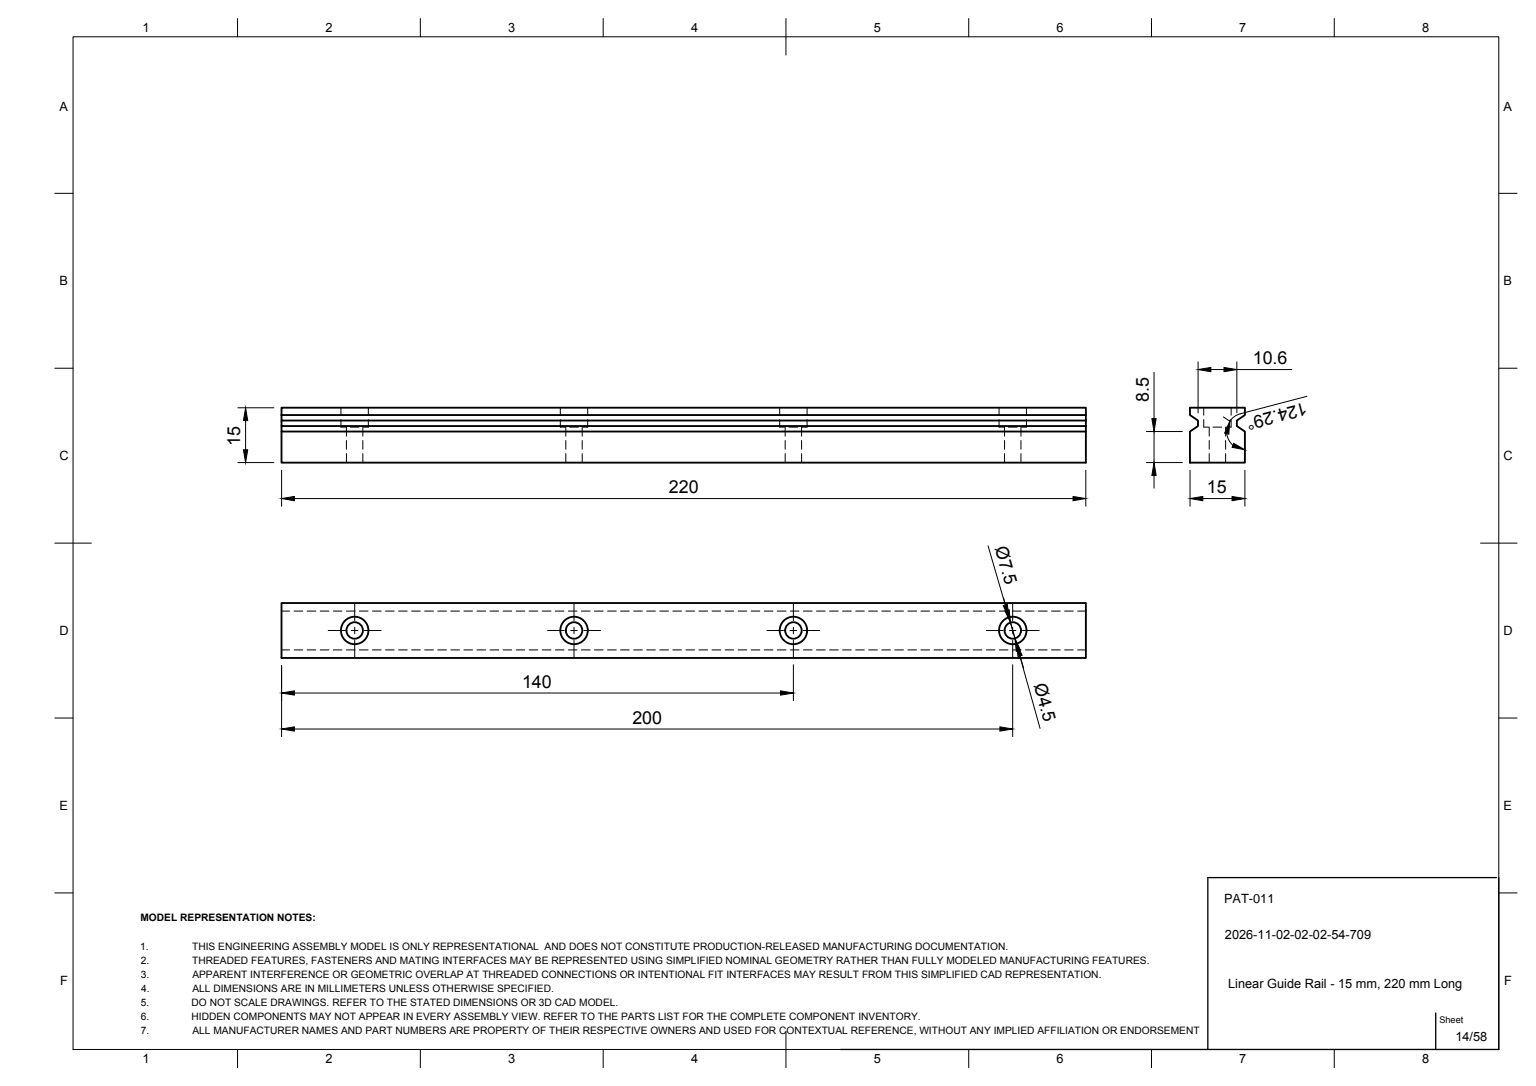
ISO-10303-21;
HEADER;
/* Generated by software containing ST-Developer
 * from STEP Tools, Inc. (www.steptools.com) 
 */

FILE_DESCRIPTION(
/* description */ ('Belt tension measurement rig'),
/* implementation_level */ '2;1');

FILE_NAME(
/* name */ 'Linear Guide Rail - 15 mm, 220 mm Long.step',
/* time_stamp */ '2026-10-28T03:24:44-07:00',
/* author */ (''),
/* organization */ (''),
/* preprocessor_version */ 'ST-DEVELOPER v20.2',
/* originating_system */ 'Autodesk Translation Framework v15.17.0.0',
/* authorisation */ '');

FILE_SCHEMA (('AUTOMOTIVE_DESIGN { 1 0 10303 214 3 1 1 }'));
ENDSEC;

DATA;
#10=MECHANICAL_DESIGN_GEOMETRIC_PRESENTATION_REPRESENTATION('',(#705),#23587);
#595=SHAPE_REPRESENTATION_RELATIONSHIP('SRR','None',#23840,#650);
#650=ADVANCED_BREP_SHAPE_REPRESENTATION('',(#775),#23538);
#705=STYLED_ITEM('',(#24204),#775);
#775=MANIFOLD_SOLID_BREP('Body1',#12210);
#895=FACE_BOUND('',#2275,.T.);
#896=FACE_BOUND('',#2278,.T.);
#897=FACE_BOUND('',#2281,.T.);
#898=FACE_BOUND('',#2284,.T.);
#899=FACE_BOUND('',#2294,.T.);
#900=FACE_BOUND('',#2295,.T.);
#901=FACE_BOUND('',#2296,.T.);
#902=FACE_BOUND('',#2297,.T.);
#903=FACE_BOUND('',#2304,.T.);
#904=FACE_BOUND('',#2305,.T.);
#905=FACE_BOUND('',#2306,.T.);
#906=FACE_BOUND('',#2307,.T.);
#1120=PLANE('',#13182);
#1121=PLANE('',#13187);
#1122=PLANE('',#13192);
#1123=PLANE('',#13197);
#1124=PLANE('',#13207);
#1125=PLANE('',#13208);
#1126=PLANE('',#13209);
#1127=PLANE('',#13210);
#1128=PLANE('',#13211);
#1129=PLANE('',#13212);
#1130=PLANE('',#13213);
#1131=PLANE('',#13214);
#1132=PLANE('',#13215);
#1133=PLANE('',#13216);
#1134=PLANE('',#13217);
#1135=PLANE('',#13218);
#1136=PLANE('',#13219);
#1137=PLANE('',#13220);
#1503=FACE_OUTER_BOUND('',#2273,.T.);
#1504=FACE_OUTER_BOUND('',#2274,.T.);
#1505=FACE_OUTER_BOUND('',#2276,.T.);
#1506=FACE_OUTER_BOUND('',#2277,.T.);
#1507=FACE_OUTER_BOUND('',#2279,.T.);
#1508=FACE_OUTER_BOUND('',#2280,.T.);
#1509=FACE_OUTER_BOUND('',#2282,.T.);
#1510=FACE_OUTER_BOUND('',#2283,.T.);
#1511=FACE_OUTER_BOUND('',#2285,.T.);
#1512=FACE_OUTER_BOUND('',#2286,.T.);
#1513=FACE_OUTER_BOUND('',#2287,.T.);
#1514=FACE_OUTER_BOUND('',#2288,.T.);
#1515=FACE_OUTER_BOUND('',#2289,.T.);
#1516=FACE_OUTER_BOUND('',#2290,.T.);
#1517=FACE_OUTER_BOUND('',#2291,.T.);
#1518=FACE_OUTER_BOUND('',#2292,.T.);
#1519=FACE_OUTER_BOUND('',#2293,.T.);
#1520=FACE_OUTER_BOUND('',#2298,.T.);
#1521=FACE_OUTER_BOUND('',#2299,.T.);
#1522=FACE_OUTER_BOUND('',#2300,.T.);
#1523=FACE_OUTER_BOUND('',#2301,.T.);
#1524=FACE_OUTER_BOUND('',#2302,.T.);
#1525=FACE_OUTER_BOUND('',#2303,.T.);
#1526=FACE_OUTER_BOUND('',#2308,.T.);
#1527=FACE_OUTER_BOUND('',#2309,.T.);
#1528=FACE_OUTER_BOUND('',#2310,.T.);
#2273=EDGE_LOOP('',(#8564,#8565,#8566,#8567));
#2274=EDGE_LOOP('',(#8568));
#2275=EDGE_LOOP('',(#8569));
#2276=EDGE_LOOP('',(#8570,#8571,#8572,#8573));
#2277=EDGE_LOOP('',(#8574));
#2278=EDGE_LOOP('',(#8575));
#2279=EDGE_LOOP('',(#8576,#8577,#8578,#8579));
#2280=EDGE_LOOP('',(#8580));
#2281=EDGE_LOOP('',(#8581));
#2282=EDGE_LOOP('',(#8582,#8583,#8584,#8585));
#2283=EDGE_LOOP('',(#8586));
#2284=EDGE_LOOP('',(#8587));
#2285=EDGE_LOOP('',(#8588,#8589,#8590,#8591));
#2286=EDGE_LOOP('',(#8592,#8593,#8594,#8595));
#2287=EDGE_LOOP('',(#8596,#8597,#8598,#8599));
#2288=EDGE_LOOP('',(#8600,#8601,#8602,#8603));
#2289=EDGE_LOOP('',(#8604,#8605,#8606,#8607));
#2290=EDGE_LOOP('',(#8608,#8609,#8610,#8611));
#2291=EDGE_LOOP('',(#8612,#8613,#8614,#8615));
#2292=EDGE_LOOP('',(#8616,#8617,#8618,#8619));
#2293=EDGE_LOOP('',(#8620,#8621,#8622,#8623));
#2294=EDGE_LOOP('',(#8624));
#2295=EDGE_LOOP('',(#8625));
#2296=EDGE_LOOP('',(#8626));
#2297=EDGE_LOOP('',(#8627));
#2298=EDGE_LOOP('',(#8628,#8629,#8630,#8631));
#2299=EDGE_LOOP('',(#8632,#8633,#8634,#8635));
#2300=EDGE_LOOP('',(#8636,#8637,#8638,#8639));
#2301=EDGE_LOOP('',(#8640,#8641,#8642,#8643));
#2302=EDGE_LOOP('',(#8644,#8645,#8646,#8647));
#2303=EDGE_LOOP('',(#8648,#8649,#8650,#8651));
#2304=EDGE_LOOP('',(#8652));
#2305=EDGE_LOOP('',(#8653));
#2306=EDGE_LOOP('',(#8654));
#2307=EDGE_LOOP('',(#8655));
#2308=EDGE_LOOP('',(#8656,#8657,#8658,#8659));
#2309=EDGE_LOOP('',(#8660,#8661,#8662,#8663,#8664,#8665,#8666,#8667,#8668,
#8669,#8670,#8671));
#2310=EDGE_LOOP('',(#8672,#8673,#8674,#8675,#8676,#8677,#8678,#8679,#8680,
#8681,#8682,#8683));
#3141=LINE('',#19312,#3892);
#3142=LINE('',#19321,#3893);
#3143=LINE('',#19330,#3894);
#3144=LINE('',#19339,#3895);
#3145=LINE('',#19347,#3896);
#3146=LINE('',#19351,#3897);
#3147=LINE('',#19355,#3898);
#3148=LINE('',#19359,#3899);
#3149=LINE('',#19363,#3900);
#3150=LINE('',#19365,#3901);
#3151=LINE('',#19367,#3902);
#3152=LINE('',#19368,#3903);
#3153=LINE('',#19371,#3904);
#3154=LINE('',#19373,#3905);
#3155=LINE('',#19374,#3906);
#3156=LINE('',#19377,#3907);
#3157=LINE('',#19379,#3908);
#3158=LINE('',#19380,#3909);
#3159=LINE('',#19383,#3910);
#3160=LINE('',#19385,#3911);
#3161=LINE('',#19386,#3912);
#3162=LINE('',#19389,#3913);
#3163=LINE('',#19391,#3914);
#3164=LINE('',#19392,#3915);
#3165=LINE('',#19395,#3916);
#3166=LINE('',#19397,#3917);
#3167=LINE('',#19398,#3918);
#3168=LINE('',#19401,#3919);
#3169=LINE('',#19403,#3920);
#3170=LINE('',#19404,#3921);
#3171=LINE('',#19407,#3922);
#3172=LINE('',#19409,#3923);
#3173=LINE('',#19410,#3924);
#3174=LINE('',#19413,#3925);
#3175=LINE('',#19415,#3926);
#3176=LINE('',#19416,#3927);
#3177=LINE('',#19419,#3928);
#3178=LINE('',#19421,#3929);
#3179=LINE('',#19422,#3930);
#3180=LINE('',#19425,#3931);
#3181=LINE('',#19427,#3932);
#3182=LINE('',#19428,#3933);
#3183=LINE('',#19430,#3934);
#3184=LINE('',#19431,#3935);
#3892=VECTOR('',#15300,0.375);
#3893=VECTOR('',#15311,0.375);
#3894=VECTOR('',#15322,0.375);
#3895=VECTOR('',#15333,0.375);
#3896=VECTOR('',#15344,0.225);
#3897=VECTOR('',#15349,0.225);
#3898=VECTOR('',#15354,0.225);
#3899=VECTOR('',#15359,0.225000000000001);
#3900=VECTOR('',#15362,1.);
#3901=VECTOR('',#15363,1.);
#3902=VECTOR('',#15364,1.);
#3903=VECTOR('',#15365,1.);
#3904=VECTOR('',#15368,1.);
#3905=VECTOR('',#15369,1.);
#3906=VECTOR('',#15370,1.);
#3907=VECTOR('',#15373,1.);
#3908=VECTOR('',#15374,1.);
#3909=VECTOR('',#15375,1.);
#3910=VECTOR('',#15378,1.);
#3911=VECTOR('',#15379,1.);
#3912=VECTOR('',#15380,1.);
#3913=VECTOR('',#15383,1.);
#3914=VECTOR('',#15384,1.);
#3915=VECTOR('',#15385,1.);
#3916=VECTOR('',#15388,1.);
#3917=VECTOR('',#15389,1.);
#3918=VECTOR('',#15390,1.);
#3919=VECTOR('',#15393,1.);
#3920=VECTOR('',#15394,1.);
#3921=VECTOR('',#15395,1.);
#3922=VECTOR('',#15398,1.);
#3923=VECTOR('',#15399,1.);
#3924=VECTOR('',#15400,1.);
#3925=VECTOR('',#15403,1.);
#3926=VECTOR('',#15404,1.);
#3927=VECTOR('',#15405,1.);
#3928=VECTOR('',#15408,1.);
#3929=VECTOR('',#15409,1.);
#3930=VECTOR('',#15410,1.);
#3931=VECTOR('',#15413,1.);
#3932=VECTOR('',#15414,1.);
#3933=VECTOR('',#15415,1.);
#3934=VECTOR('',#15418,1.);
#3935=VECTOR('',#15419,1.);
#4606=CIRCLE('',#13180,0.375);
#4607=CIRCLE('',#13181,0.375);
#4608=CIRCLE('',#13183,0.225);
#4609=CIRCLE('',#13185,0.375);
#4610=CIRCLE('',#13186,0.375);
#4611=CIRCLE('',#13188,0.225);
#4612=CIRCLE('',#13190,0.375);
#4613=CIRCLE('',#13191,0.375);
#4614=CIRCLE('',#13193,0.225);
#4615=CIRCLE('',#13195,0.375);
#4616=CIRCLE('',#13196,0.375);
#4617=CIRCLE('',#13198,0.225000000000001);
#4618=CIRCLE('',#13200,0.225);
#4619=CIRCLE('',#13202,0.225);
#4620=CIRCLE('',#13204,0.225);
#4621=CIRCLE('',#13206,0.225000000000001);
#5444=VERTEX_POINT('',#19309);
#5445=VERTEX_POINT('',#19311);
#5446=VERTEX_POINT('',#19315);
#5447=VERTEX_POINT('',#19318);
#5448=VERTEX_POINT('',#19320);
#5449=VERTEX_POINT('',#19324);
#5450=VERTEX_POINT('',#19327);
#5451=VERTEX_POINT('',#19329);
#5452=VERTEX_POINT('',#19333);
#5453=VERTEX_POINT('',#19336);
#5454=VERTEX_POINT('',#19338);
#5455=VERTEX_POINT('',#19342);
#5456=VERTEX_POINT('',#19345);
#5457=VERTEX_POINT('',#19349);
#5458=VERTEX_POINT('',#19353);
#5459=VERTEX_POINT('',#19357);
#5460=VERTEX_POINT('',#19361);
#5461=VERTEX_POINT('',#19362);
#5462=VERTEX_POINT('',#19364);
#5463=VERTEX_POINT('',#19366);
#5464=VERTEX_POINT('',#19370);
#5465=VERTEX_POINT('',#19372);
#5466=VERTEX_POINT('',#19376);
#5467=VERTEX_POINT('',#19378);
#5468=VERTEX_POINT('',#19382);
#5469=VERTEX_POINT('',#19384);
#5470=VERTEX_POINT('',#19388);
#5471=VERTEX_POINT('',#19390);
#5472=VERTEX_POINT('',#19394);
#5473=VERTEX_POINT('',#19396);
#5474=VERTEX_POINT('',#19400);
#5475=VERTEX_POINT('',#19402);
#5476=VERTEX_POINT('',#19406);
#5477=VERTEX_POINT('',#19408);
#5478=VERTEX_POINT('',#19412);
#5479=VERTEX_POINT('',#19414);
#5480=VERTEX_POINT('',#19418);
#5481=VERTEX_POINT('',#19420);
#5482=VERTEX_POINT('',#19424);
#5483=VERTEX_POINT('',#19426);
#6641=EDGE_CURVE('',#5444,#5444,#4606,.T.);
#6642=EDGE_CURVE('',#5444,#5445,#3141,.T.);
#6643=EDGE_CURVE('',#5445,#5445,#4607,.T.);
#6644=EDGE_CURVE('',#5446,#5446,#4608,.T.);
#6645=EDGE_CURVE('',#5447,#5447,#4609,.T.);
#6646=EDGE_CURVE('',#5447,#5448,#3142,.T.);
#6647=EDGE_CURVE('',#5448,#5448,#4610,.T.);
#6648=EDGE_CURVE('',#5449,#5449,#4611,.T.);
#6649=EDGE_CURVE('',#5450,#5450,#4612,.T.);
#6650=EDGE_CURVE('',#5450,#5451,#3143,.T.);
#6651=EDGE_CURVE('',#5451,#5451,#4613,.T.);
#6652=EDGE_CURVE('',#5452,#5452,#4614,.T.);
#6653=EDGE_CURVE('',#5453,#5453,#4615,.T.);
#6654=EDGE_CURVE('',#5453,#5454,#3144,.T.);
#6655=EDGE_CURVE('',#5454,#5454,#4616,.T.);
#6656=EDGE_CURVE('',#5455,#5455,#4617,.T.);
#6657=EDGE_CURVE('',#5456,#5456,#4618,.T.);
#6658=EDGE_CURVE('',#5456,#5446,#3145,.T.);
#6659=EDGE_CURVE('',#5457,#5457,#4619,.T.);
#6660=EDGE_CURVE('',#5457,#5449,#3146,.T.);
#6661=EDGE_CURVE('',#5458,#5458,#4620,.T.);
#6662=EDGE_CURVE('',#5458,#5452,#3147,.T.);
#6663=EDGE_CURVE('',#5459,#5459,#4621,.T.);
#6664=EDGE_CURVE('',#5459,#5455,#3148,.T.);
#6665=EDGE_CURVE('',#5460,#5461,#3149,.T.);
#6666=EDGE_CURVE('',#5461,#5462,#3150,.T.);
#6667=EDGE_CURVE('',#5463,#5462,#3151,.T.);
#6668=EDGE_CURVE('',#5460,#5463,#3152,.T.);
#6669=EDGE_CURVE('',#5464,#5460,#3153,.T.);
#6670=EDGE_CURVE('',#5465,#5463,#3154,.T.);
#6671=EDGE_CURVE('',#5464,#5465,#3155,.T.);
#6672=EDGE_CURVE('',#5466,#5464,#3156,.T.);
#6673=EDGE_CURVE('',#5467,#5465,#3157,.T.);
#6674=EDGE_CURVE('',#5466,#5467,#3158,.T.);
#6675=EDGE_CURVE('',#5468,#5466,#3159,.T.);
#6676=EDGE_CURVE('',#5469,#5467,#3160,.T.);
#6677=EDGE_CURVE('',#5468,#5469,#3161,.T.);
#6678=EDGE_CURVE('',#5470,#5468,#3162,.T.);
#6679=EDGE_CURVE('',#5471,#5469,#3163,.T.);
#6680=EDGE_CURVE('',#5470,#5471,#3164,.T.);
#6681=EDGE_CURVE('',#5472,#5470,#3165,.T.);
#6682=EDGE_CURVE('',#5473,#5471,#3166,.T.);
#6683=EDGE_CURVE('',#5472,#5473,#3167,.T.);
#6684=EDGE_CURVE('',#5474,#5472,#3168,.T.);
#6685=EDGE_CURVE('',#5475,#5473,#3169,.T.);
#6686=EDGE_CURVE('',#5474,#5475,#3170,.T.);
#6687=EDGE_CURVE('',#5476,#5474,#3171,.T.);
#6688=EDGE_CURVE('',#5477,#5475,#3172,.T.);
#6689=EDGE_CURVE('',#5476,#5477,#3173,.T.);
#6690=EDGE_CURVE('',#5478,#5476,#3174,.T.);
#6691=EDGE_CURVE('',#5479,#5477,#3175,.T.);
#6692=EDGE_CURVE('',#5478,#5479,#3176,.T.);
#6693=EDGE_CURVE('',#5480,#5478,#3177,.T.);
#6694=EDGE_CURVE('',#5481,#5479,#3178,.T.);
#6695=EDGE_CURVE('',#5480,#5481,#3179,.T.);
#6696=EDGE_CURVE('',#5482,#5480,#3180,.T.);
#6697=EDGE_CURVE('',#5483,#5481,#3181,.T.);
#6698=EDGE_CURVE('',#5482,#5483,#3182,.T.);
#6699=EDGE_CURVE('',#5461,#5482,#3183,.T.);
#6700=EDGE_CURVE('',#5462,#5483,#3184,.T.);
#8564=ORIENTED_EDGE('',*,*,#6641,.F.);
#8565=ORIENTED_EDGE('',*,*,#6642,.T.);
#8566=ORIENTED_EDGE('',*,*,#6643,.F.);
#8567=ORIENTED_EDGE('',*,*,#6642,.F.);
#8568=ORIENTED_EDGE('',*,*,#6641,.T.);
#8569=ORIENTED_EDGE('',*,*,#6644,.F.);
#8570=ORIENTED_EDGE('',*,*,#6645,.F.);
#8571=ORIENTED_EDGE('',*,*,#6646,.T.);
#8572=ORIENTED_EDGE('',*,*,#6647,.F.);
#8573=ORIENTED_EDGE('',*,*,#6646,.F.);
#8574=ORIENTED_EDGE('',*,*,#6645,.T.);
#8575=ORIENTED_EDGE('',*,*,#6648,.F.);
#8576=ORIENTED_EDGE('',*,*,#6649,.F.);
#8577=ORIENTED_EDGE('',*,*,#6650,.T.);
#8578=ORIENTED_EDGE('',*,*,#6651,.F.);
#8579=ORIENTED_EDGE('',*,*,#6650,.F.);
#8580=ORIENTED_EDGE('',*,*,#6649,.T.);
#8581=ORIENTED_EDGE('',*,*,#6652,.F.);
#8582=ORIENTED_EDGE('',*,*,#6653,.F.);
#8583=ORIENTED_EDGE('',*,*,#6654,.T.);
#8584=ORIENTED_EDGE('',*,*,#6655,.F.);
#8585=ORIENTED_EDGE('',*,*,#6654,.F.);
#8586=ORIENTED_EDGE('',*,*,#6653,.T.);
#8587=ORIENTED_EDGE('',*,*,#6656,.F.);
#8588=ORIENTED_EDGE('',*,*,#6657,.F.);
#8589=ORIENTED_EDGE('',*,*,#6658,.T.);
#8590=ORIENTED_EDGE('',*,*,#6644,.T.);
#8591=ORIENTED_EDGE('',*,*,#6658,.F.);
#8592=ORIENTED_EDGE('',*,*,#6659,.F.);
#8593=ORIENTED_EDGE('',*,*,#6660,.T.);
#8594=ORIENTED_EDGE('',*,*,#6648,.T.);
#8595=ORIENTED_EDGE('',*,*,#6660,.F.);
#8596=ORIENTED_EDGE('',*,*,#6661,.F.);
#8597=ORIENTED_EDGE('',*,*,#6662,.T.);
#8598=ORIENTED_EDGE('',*,*,#6652,.T.);
#8599=ORIENTED_EDGE('',*,*,#6662,.F.);
#8600=ORIENTED_EDGE('',*,*,#6663,.F.);
#8601=ORIENTED_EDGE('',*,*,#6664,.T.);
#8602=ORIENTED_EDGE('',*,*,#6656,.T.);
#8603=ORIENTED_EDGE('',*,*,#6664,.F.);
#8604=ORIENTED_EDGE('',*,*,#6665,.T.);
#8605=ORIENTED_EDGE('',*,*,#6666,.T.);
#8606=ORIENTED_EDGE('',*,*,#6667,.F.);
#8607=ORIENTED_EDGE('',*,*,#6668,.F.);
#8608=ORIENTED_EDGE('',*,*,#6669,.T.);
#8609=ORIENTED_EDGE('',*,*,#6668,.T.);
#8610=ORIENTED_EDGE('',*,*,#6670,.F.);
#8611=ORIENTED_EDGE('',*,*,#6671,.F.);
#8612=ORIENTED_EDGE('',*,*,#6672,.T.);
#8613=ORIENTED_EDGE('',*,*,#6671,.T.);
#8614=ORIENTED_EDGE('',*,*,#6673,.F.);
#8615=ORIENTED_EDGE('',*,*,#6674,.F.);
#8616=ORIENTED_EDGE('',*,*,#6675,.T.);
#8617=ORIENTED_EDGE('',*,*,#6674,.T.);
#8618=ORIENTED_EDGE('',*,*,#6676,.F.);
#8619=ORIENTED_EDGE('',*,*,#6677,.F.);
#8620=ORIENTED_EDGE('',*,*,#6678,.T.);
#8621=ORIENTED_EDGE('',*,*,#6677,.T.);
#8622=ORIENTED_EDGE('',*,*,#6679,.F.);
#8623=ORIENTED_EDGE('',*,*,#6680,.F.);
#8624=ORIENTED_EDGE('',*,*,#6655,.T.);
#8625=ORIENTED_EDGE('',*,*,#6651,.T.);
#8626=ORIENTED_EDGE('',*,*,#6647,.T.);
#8627=ORIENTED_EDGE('',*,*,#6643,.T.);
#8628=ORIENTED_EDGE('',*,*,#6681,.T.);
#8629=ORIENTED_EDGE('',*,*,#6680,.T.);
#8630=ORIENTED_EDGE('',*,*,#6682,.F.);
#8631=ORIENTED_EDGE('',*,*,#6683,.F.);
#8632=ORIENTED_EDGE('',*,*,#6684,.T.);
#8633=ORIENTED_EDGE('',*,*,#6683,.T.);
#8634=ORIENTED_EDGE('',*,*,#6685,.F.);
#8635=ORIENTED_EDGE('',*,*,#6686,.F.);
#8636=ORIENTED_EDGE('',*,*,#6687,.T.);
#8637=ORIENTED_EDGE('',*,*,#6686,.T.);
#8638=ORIENTED_EDGE('',*,*,#6688,.F.);
#8639=ORIENTED_EDGE('',*,*,#6689,.F.);
#8640=ORIENTED_EDGE('',*,*,#6690,.T.);
#8641=ORIENTED_EDGE('',*,*,#6689,.T.);
#8642=ORIENTED_EDGE('',*,*,#6691,.F.);
#8643=ORIENTED_EDGE('',*,*,#6692,.F.);
#8644=ORIENTED_EDGE('',*,*,#6693,.T.);
#8645=ORIENTED_EDGE('',*,*,#6692,.T.);
#8646=ORIENTED_EDGE('',*,*,#6694,.F.);
#8647=ORIENTED_EDGE('',*,*,#6695,.F.);
#8648=ORIENTED_EDGE('',*,*,#6696,.T.);
#8649=ORIENTED_EDGE('',*,*,#6695,.T.);
#8650=ORIENTED_EDGE('',*,*,#6697,.F.);
#8651=ORIENTED_EDGE('',*,*,#6698,.F.);
#8652=ORIENTED_EDGE('',*,*,#6657,.T.);
#8653=ORIENTED_EDGE('',*,*,#6659,.T.);
#8654=ORIENTED_EDGE('',*,*,#6661,.T.);
#8655=ORIENTED_EDGE('',*,*,#6663,.T.);
#8656=ORIENTED_EDGE('',*,*,#6699,.T.);
#8657=ORIENTED_EDGE('',*,*,#6698,.T.);
#8658=ORIENTED_EDGE('',*,*,#6700,.F.);
#8659=ORIENTED_EDGE('',*,*,#6666,.F.);
#8660=ORIENTED_EDGE('',*,*,#6700,.T.);
#8661=ORIENTED_EDGE('',*,*,#6697,.T.);
#8662=ORIENTED_EDGE('',*,*,#6694,.T.);
#8663=ORIENTED_EDGE('',*,*,#6691,.T.);
#8664=ORIENTED_EDGE('',*,*,#6688,.T.);
#8665=ORIENTED_EDGE('',*,*,#6685,.T.);
#8666=ORIENTED_EDGE('',*,*,#6682,.T.);
#8667=ORIENTED_EDGE('',*,*,#6679,.T.);
#8668=ORIENTED_EDGE('',*,*,#6676,.T.);
#8669=ORIENTED_EDGE('',*,*,#6673,.T.);
#8670=ORIENTED_EDGE('',*,*,#6670,.T.);
#8671=ORIENTED_EDGE('',*,*,#6667,.T.);
#8672=ORIENTED_EDGE('',*,*,#6699,.F.);
#8673=ORIENTED_EDGE('',*,*,#6665,.F.);
#8674=ORIENTED_EDGE('',*,*,#6669,.F.);
#8675=ORIENTED_EDGE('',*,*,#6672,.F.);
#8676=ORIENTED_EDGE('',*,*,#6675,.F.);
#8677=ORIENTED_EDGE('',*,*,#6678,.F.);
#8678=ORIENTED_EDGE('',*,*,#6681,.F.);
#8679=ORIENTED_EDGE('',*,*,#6684,.F.);
#8680=ORIENTED_EDGE('',*,*,#6687,.F.);
#8681=ORIENTED_EDGE('',*,*,#6690,.F.);
#8682=ORIENTED_EDGE('',*,*,#6693,.F.);
#8683=ORIENTED_EDGE('',*,*,#6696,.F.);
#11226=CYLINDRICAL_SURFACE('',#13179,0.375);
#11227=CYLINDRICAL_SURFACE('',#13184,0.375);
#11228=CYLINDRICAL_SURFACE('',#13189,0.375);
#11229=CYLINDRICAL_SURFACE('',#13194,0.375);
#11230=CYLINDRICAL_SURFACE('',#13199,0.225);
#11231=CYLINDRICAL_SURFACE('',#13201,0.225);
#11232=CYLINDRICAL_SURFACE('',#13203,0.225);
#11233=CYLINDRICAL_SURFACE('',#13205,0.225000000000001);
#11644=ADVANCED_FACE('',(#1503),#11226,.F.);
#11645=ADVANCED_FACE('',(#1504,#895),#1120,.T.);
#11646=ADVANCED_FACE('',(#1505),#11227,.F.);
#11647=ADVANCED_FACE('',(#1506,#896),#1121,.T.);
#11648=ADVANCED_FACE('',(#1507),#11228,.F.);
#11649=ADVANCED_FACE('',(#1508,#897),#1122,.T.);
#11650=ADVANCED_FACE('',(#1509),#11229,.F.);
#11651=ADVANCED_FACE('',(#1510,#898),#1123,.T.);
#11652=ADVANCED_FACE('',(#1511),#11230,.F.);
#11653=ADVANCED_FACE('',(#1512),#11231,.F.);
#11654=ADVANCED_FACE('',(#1513),#11232,.F.);
#11655=ADVANCED_FACE('',(#1514),#11233,.F.);
#11656=ADVANCED_FACE('',(#1515),#1124,.T.);
#11657=ADVANCED_FACE('',(#1516),#1125,.T.);
#11658=ADVANCED_FACE('',(#1517),#1126,.T.);
#11659=ADVANCED_FACE('',(#1518),#1127,.T.);
#11660=ADVANCED_FACE('',(#1519,#899,#900,#901,#902),#1128,.T.);
#11661=ADVANCED_FACE('',(#1520),#1129,.T.);
#11662=ADVANCED_FACE('',(#1521),#1130,.T.);
#11663=ADVANCED_FACE('',(#1522),#1131,.T.);
#11664=ADVANCED_FACE('',(#1523),#1132,.T.);
#11665=ADVANCED_FACE('',(#1524),#1133,.T.);
#11666=ADVANCED_FACE('',(#1525,#903,#904,#905,#906),#1134,.T.);
#11667=ADVANCED_FACE('',(#1526),#1135,.T.);
#11668=ADVANCED_FACE('',(#1527),#1136,.T.);
#11669=ADVANCED_FACE('',(#1528),#1137,.F.);
#12210=CLOSED_SHELL('',(#11644,#11645,#11646,#11647,#11648,#11649,#11650,
#11651,#11652,#11653,#11654,#11655,#11656,#11657,#11658,#11659,#11660,#11661,
#11662,#11663,#11664,#11665,#11666,#11667,#11668,#11669));
#13178=AXIS2_PLACEMENT_3D('',#19307,#15294,#15295);
#13179=AXIS2_PLACEMENT_3D('',#19308,#15296,#15297);
#13180=AXIS2_PLACEMENT_3D('',#19310,#15298,#15299);
#13181=AXIS2_PLACEMENT_3D('',#19313,#15301,#15302);
#13182=AXIS2_PLACEMENT_3D('',#19314,#15303,#15304);
#13183=AXIS2_PLACEMENT_3D('',#19316,#15305,#15306);
#13184=AXIS2_PLACEMENT_3D('',#19317,#15307,#15308);
#13185=AXIS2_PLACEMENT_3D('',#19319,#15309,#15310);
#13186=AXIS2_PLACEMENT_3D('',#19322,#15312,#15313);
#13187=AXIS2_PLACEMENT_3D('',#19323,#15314,#15315);
#13188=AXIS2_PLACEMENT_3D('',#19325,#15316,#15317);
#13189=AXIS2_PLACEMENT_3D('',#19326,#15318,#15319);
#13190=AXIS2_PLACEMENT_3D('',#19328,#15320,#15321);
#13191=AXIS2_PLACEMENT_3D('',#19331,#15323,#15324);
#13192=AXIS2_PLACEMENT_3D('',#19332,#15325,#15326);
#13193=AXIS2_PLACEMENT_3D('',#19334,#15327,#15328);
#13194=AXIS2_PLACEMENT_3D('',#19335,#15329,#15330);
#13195=AXIS2_PLACEMENT_3D('',#19337,#15331,#15332);
#13196=AXIS2_PLACEMENT_3D('',#19340,#15334,#15335);
#13197=AXIS2_PLACEMENT_3D('',#19341,#15336,#15337);
#13198=AXIS2_PLACEMENT_3D('',#19343,#15338,#15339);
#13199=AXIS2_PLACEMENT_3D('',#19344,#15340,#15341);
#13200=AXIS2_PLACEMENT_3D('',#19346,#15342,#15343);
#13201=AXIS2_PLACEMENT_3D('',#19348,#15345,#15346);
#13202=AXIS2_PLACEMENT_3D('',#19350,#15347,#15348);
#13203=AXIS2_PLACEMENT_3D('',#19352,#15350,#15351);
#13204=AXIS2_PLACEMENT_3D('',#19354,#15352,#15353);
#13205=AXIS2_PLACEMENT_3D('',#19356,#15355,#15356);
#13206=AXIS2_PLACEMENT_3D('',#19358,#15357,#15358);
#13207=AXIS2_PLACEMENT_3D('',#19360,#15360,#15361);
#13208=AXIS2_PLACEMENT_3D('',#19369,#15366,#15367);
#13209=AXIS2_PLACEMENT_3D('',#19375,#15371,#15372);
#13210=AXIS2_PLACEMENT_3D('',#19381,#15376,#15377);
#13211=AXIS2_PLACEMENT_3D('',#19387,#15381,#15382);
#13212=AXIS2_PLACEMENT_3D('',#19393,#15386,#15387);
#13213=AXIS2_PLACEMENT_3D('',#19399,#15391,#15392);
#13214=AXIS2_PLACEMENT_3D('',#19405,#15396,#15397);
#13215=AXIS2_PLACEMENT_3D('',#19411,#15401,#15402);
#13216=AXIS2_PLACEMENT_3D('',#19417,#15406,#15407);
#13217=AXIS2_PLACEMENT_3D('',#19423,#15411,#15412);
#13218=AXIS2_PLACEMENT_3D('',#19429,#15416,#15417);
#13219=AXIS2_PLACEMENT_3D('',#19432,#15420,#15421);
#13220=AXIS2_PLACEMENT_3D('',#19433,#15422,#15423);
#15294=DIRECTION('axis',(0.,0.,1.));
#15295=DIRECTION('refdir',(1.,0.,0.));
#15296=DIRECTION('center_axis',(0.,0.,1.));
#15297=DIRECTION('ref_axis',(1.,0.,0.));
#15298=DIRECTION('center_axis',(0.,0.,1.));
#15299=DIRECTION('ref_axis',(1.,0.,0.));
#15300=DIRECTION('',(0.,0.,1.));
#15301=DIRECTION('center_axis',(0.,0.,-1.));
#15302=DIRECTION('ref_axis',(1.,0.,0.));
#15303=DIRECTION('center_axis',(0.,0.,1.));
#15304=DIRECTION('ref_axis',(1.,0.,0.));
#15305=DIRECTION('center_axis',(0.,0.,1.));
#15306=DIRECTION('ref_axis',(1.,0.,0.));
#15307=DIRECTION('center_axis',(0.,0.,1.));
#15308=DIRECTION('ref_axis',(1.,0.,0.));
#15309=DIRECTION('center_axis',(0.,0.,1.));
#15310=DIRECTION('ref_axis',(1.,0.,0.));
#15311=DIRECTION('',(0.,0.,1.));
#15312=DIRECTION('center_axis',(0.,0.,-1.));
#15313=DIRECTION('ref_axis',(1.,0.,0.));
#15314=DIRECTION('center_axis',(0.,0.,1.));
#15315=DIRECTION('ref_axis',(1.,0.,0.));
#15316=DIRECTION('center_axis',(0.,0.,1.));
#15317=DIRECTION('ref_axis',(1.,0.,0.));
#15318=DIRECTION('center_axis',(0.,0.,1.));
#15319=DIRECTION('ref_axis',(1.,0.,0.));
#15320=DIRECTION('center_axis',(0.,0.,1.));
#15321=DIRECTION('ref_axis',(1.,0.,0.));
#15322=DIRECTION('',(0.,0.,1.));
#15323=DIRECTION('center_axis',(0.,0.,-1.));
#15324=DIRECTION('ref_axis',(1.,0.,0.));
#15325=DIRECTION('center_axis',(0.,0.,1.));
#15326=DIRECTION('ref_axis',(1.,0.,0.));
#15327=DIRECTION('center_axis',(0.,0.,1.));
#15328=DIRECTION('ref_axis',(1.,0.,0.));
#15329=DIRECTION('center_axis',(0.,0.,1.));
#15330=DIRECTION('ref_axis',(1.,0.,0.));
#15331=DIRECTION('center_axis',(0.,0.,1.));
#15332=DIRECTION('ref_axis',(1.,0.,0.));
#15333=DIRECTION('',(0.,0.,1.));
#15334=DIRECTION('center_axis',(0.,0.,-1.));
#15335=DIRECTION('ref_axis',(1.,0.,0.));
#15336=DIRECTION('center_axis',(0.,0.,1.));
#15337=DIRECTION('ref_axis',(1.,0.,0.));
#15338=DIRECTION('center_axis',(0.,0.,1.));
#15339=DIRECTION('ref_axis',(1.,0.,0.));
#15340=DIRECTION('center_axis',(0.,0.,1.));
#15341=DIRECTION('ref_axis',(1.,0.,0.));
#15342=DIRECTION('center_axis',(0.,0.,1.));
#15343=DIRECTION('ref_axis',(1.,0.,0.));
#15344=DIRECTION('',(0.,0.,1.));
#15345=DIRECTION('center_axis',(0.,0.,1.));
#15346=DIRECTION('ref_axis',(1.,0.,0.));
#15347=DIRECTION('center_axis',(0.,0.,1.));
#15348=DIRECTION('ref_axis',(1.,0.,0.));
#15349=DIRECTION('',(0.,0.,1.));
#15350=DIRECTION('center_axis',(0.,0.,1.));
#15351=DIRECTION('ref_axis',(1.,0.,0.));
#15352=DIRECTION('center_axis',(0.,0.,1.));
#15353=DIRECTION('ref_axis',(1.,0.,0.));
#15354=DIRECTION('',(0.,0.,1.));
#15355=DIRECTION('center_axis',(0.,0.,1.));
#15356=DIRECTION('ref_axis',(1.,0.,0.));
#15357=DIRECTION('center_axis',(0.,0.,1.));
#15358=DIRECTION('ref_axis',(1.,0.,0.));
#15359=DIRECTION('',(0.,0.,1.));
#15360=DIRECTION('center_axis',(0.,-0.56333682464151,0.826227342807548));
#15361=DIRECTION('ref_axis',(0.,-0.826227342807548,-0.56333682464151));
#15362=DIRECTION('',(0.,-0.826227342807548,-0.56333682464151));
#15363=DIRECTION('',(1.,0.,0.));
#15364=DIRECTION('',(0.,-0.826227342807548,-0.56333682464151));
#15365=DIRECTION('',(1.,0.,0.));
#15366=DIRECTION('center_axis',(0.,-1.,0.));
#15367=DIRECTION('ref_axis',(0.,0.,-1.));
#15368=DIRECTION('',(0.,0.,-1.));
#15369=DIRECTION('',(0.,0.,-1.));
#15370=DIRECTION('',(1.,0.,0.));
#15371=DIRECTION('center_axis',(0.,-0.56333682464151,-0.826227342807548));
#15372=DIRECTION('ref_axis',(0.,0.826227342807548,-0.56333682464151));
#15373=DIRECTION('',(0.,0.826227342807548,-0.56333682464151));
#15374=DIRECTION('',(0.,0.826227342807548,-0.56333682464151));
#15375=DIRECTION('',(1.,0.,0.));
#15376=DIRECTION('center_axis',(0.,-1.,0.));
#15377=DIRECTION('ref_axis',(0.,0.,-1.));
#15378=DIRECTION('',(0.,0.,-1.));
#15379=DIRECTION('',(0.,0.,-1.));
#15380=DIRECTION('',(1.,0.,0.));
#15381=DIRECTION('center_axis',(0.,0.,1.));
#15382=DIRECTION('ref_axis',(0.,-1.,0.));
#15383=DIRECTION('',(0.,-1.,0.));
#15384=DIRECTION('',(0.,-1.,0.));
#15385=DIRECTION('',(1.,0.,0.));
#15386=DIRECTION('center_axis',(0.,1.,0.));
#15387=DIRECTION('ref_axis',(0.,0.,1.));
#15388=DIRECTION('',(0.,0.,1.));
#15389=DIRECTION('',(0.,0.,1.));
#15390=DIRECTION('',(1.,0.,0.));
#15391=DIRECTION('center_axis',(0.,0.56333682464151,-0.826227342807548));
#15392=DIRECTION('ref_axis',(0.,0.826227342807548,0.56333682464151));
#15393=DIRECTION('',(0.,0.826227342807548,0.56333682464151));
#15394=DIRECTION('',(0.,0.826227342807548,0.56333682464151));
#15395=DIRECTION('',(1.,0.,0.));
#15396=DIRECTION('center_axis',(0.,1.,0.));
#15397=DIRECTION('ref_axis',(0.,0.,1.));
#15398=DIRECTION('',(0.,0.,1.));
#15399=DIRECTION('',(0.,0.,1.));
#15400=DIRECTION('',(1.,0.,0.));
#15401=DIRECTION('center_axis',(0.,0.56333682464151,0.826227342807548));
#15402=DIRECTION('ref_axis',(0.,-0.826227342807548,0.56333682464151));
#15403=DIRECTION('',(0.,-0.826227342807548,0.56333682464151));
#15404=DIRECTION('',(0.,-0.826227342807548,0.56333682464151));
#15405=DIRECTION('',(1.,0.,0.));
#15406=DIRECTION('center_axis',(0.,1.,0.));
#15407=DIRECTION('ref_axis',(0.,0.,1.));
#15408=DIRECTION('',(0.,0.,1.));
#15409=DIRECTION('',(0.,0.,1.));
#15410=DIRECTION('',(1.,0.,0.));
#15411=DIRECTION('center_axis',(0.,0.,-1.));
#15412=DIRECTION('ref_axis',(0.,1.,0.));
#15413=DIRECTION('',(0.,1.,0.));
#15414=DIRECTION('',(0.,1.,0.));
#15415=DIRECTION('',(1.,0.,0.));
#15416=DIRECTION('center_axis',(0.,-1.,0.));
#15417=DIRECTION('ref_axis',(0.,0.,-1.));
#15418=DIRECTION('',(0.,0.,-1.));
#15419=DIRECTION('',(0.,0.,-1.));
#15420=DIRECTION('center_axis',(1.,0.,0.));
#15421=DIRECTION('ref_axis',(0.,0.,-1.));
#15422=DIRECTION('center_axis',(1.,0.,0.));
#15423=DIRECTION('ref_axis',(0.,0.,-1.));
#19307=CARTESIAN_POINT('',(0.,0.,0.));
#19308=CARTESIAN_POINT('Origin',(14.,0.,0.97));
#19309=CARTESIAN_POINT('',(13.625,-4.59242549680257E-17,0.97));
#19310=CARTESIAN_POINT('Origin',(14.,0.,0.97));
#19311=CARTESIAN_POINT('',(13.625,4.59242549680257E-17,1.5));
#19312=CARTESIAN_POINT('',(13.625,-4.59242549680257E-17,0.97));
#19313=CARTESIAN_POINT('Origin',(14.,0.,1.5));
#19314=CARTESIAN_POINT('Origin',(14.,0.,0.97));
#19315=CARTESIAN_POINT('',(13.775,-2.75545529808154E-17,0.97));
#19316=CARTESIAN_POINT('Origin',(14.,0.,0.97));
#19317=CARTESIAN_POINT('Origin',(8.,0.,0.97));
#19318=CARTESIAN_POINT('',(7.625,-4.59242549680257E-17,0.97));
#19319=CARTESIAN_POINT('Origin',(8.,0.,0.97));
#19320=CARTESIAN_POINT('',(7.625,4.59242549680257E-17,1.5));
#19321=CARTESIAN_POINT('',(7.625,-4.59242549680257E-17,0.97));
#19322=CARTESIAN_POINT('Origin',(8.,0.,1.5));
#19323=CARTESIAN_POINT('Origin',(8.,0.,0.97));
#19324=CARTESIAN_POINT('',(7.775,-2.75545529808154E-17,0.97));
#19325=CARTESIAN_POINT('Origin',(8.,0.,0.97));
#19326=CARTESIAN_POINT('Origin',(2.,0.,0.97));
#19327=CARTESIAN_POINT('',(1.625,-4.59242549680257E-17,0.97));
#19328=CARTESIAN_POINT('Origin',(2.,0.,0.97));
#19329=CARTESIAN_POINT('',(1.625,4.59242549680257E-17,1.5));
#19330=CARTESIAN_POINT('',(1.625,-4.59242549680257E-17,0.97));
#19331=CARTESIAN_POINT('Origin',(2.,0.,1.5));
#19332=CARTESIAN_POINT('Origin',(2.,0.,0.97));
#19333=CARTESIAN_POINT('',(1.775,-2.75545529808155E-17,0.97));
#19334=CARTESIAN_POINT('Origin',(2.,0.,0.97));
#19335=CARTESIAN_POINT('Origin',(20.,0.,0.97));
#19336=CARTESIAN_POINT('',(19.625,-4.59242549680257E-17,0.97));
#19337=CARTESIAN_POINT('Origin',(20.,0.,0.97));
#19338=CARTESIAN_POINT('',(19.625,4.59242549680257E-17,1.5));
#19339=CARTESIAN_POINT('',(19.625,-4.59242549680257E-17,0.97));
#19340=CARTESIAN_POINT('Origin',(20.,0.,1.5));
#19341=CARTESIAN_POINT('Origin',(20.,0.,0.97));
#19342=CARTESIAN_POINT('',(19.775,-2.75545529808156E-17,0.97));
#19343=CARTESIAN_POINT('Origin',(20.,0.,0.97));
#19344=CARTESIAN_POINT('Origin',(14.,0.,-0.1));
#19345=CARTESIAN_POINT('',(13.775,-2.75545529808154E-17,0.));
#19346=CARTESIAN_POINT('Origin',(14.,0.,0.));
#19347=CARTESIAN_POINT('',(13.775,-2.75545529808154E-17,-0.1));
#19348=CARTESIAN_POINT('Origin',(8.,0.,-0.1));
#19349=CARTESIAN_POINT('',(7.775,-2.75545529808154E-17,0.));
#19350=CARTESIAN_POINT('Origin',(8.,0.,0.));
#19351=CARTESIAN_POINT('',(7.775,-2.75545529808154E-17,-0.1));
#19352=CARTESIAN_POINT('Origin',(2.,0.,-0.1));
#19353=CARTESIAN_POINT('',(1.775,-2.75545529808155E-17,0.));
#19354=CARTESIAN_POINT('Origin',(2.,0.,0.));
#19355=CARTESIAN_POINT('',(1.775,-2.75545529808155E-17,-0.1));
#19356=CARTESIAN_POINT('Origin',(20.,0.,-0.1));
#19357=CARTESIAN_POINT('',(19.775,-2.75545529808156E-17,0.));
#19358=CARTESIAN_POINT('Origin',(20.,0.,0.));
#19359=CARTESIAN_POINT('',(19.775,-2.75545529808156E-17,-0.1));
#19360=CARTESIAN_POINT('Origin',(0.,-0.53,1.));
#19361=CARTESIAN_POINT('',(0.,-0.53,1.));
#19362=CARTESIAN_POINT('',(0.,-0.75,0.85));
#19363=CARTESIAN_POINT('',(0.,-0.53,1.));
#19364=CARTESIAN_POINT('',(22.,-0.75,0.85));
#19365=CARTESIAN_POINT('',(0.,-0.75,0.85));
#19366=CARTESIAN_POINT('',(22.,-0.53,1.));
#19367=CARTESIAN_POINT('',(22.,-0.53,1.));
#19368=CARTESIAN_POINT('',(0.,-0.53,1.));
#19369=CARTESIAN_POINT('Origin',(0.,-0.53,1.15));
#19370=CARTESIAN_POINT('',(0.,-0.53,1.15));
#19371=CARTESIAN_POINT('',(0.,-0.53,1.15));
#19372=CARTESIAN_POINT('',(22.,-0.53,1.15));
#19373=CARTESIAN_POINT('',(22.,-0.53,1.15));
#19374=CARTESIAN_POINT('',(0.,-0.53,1.15));
#19375=CARTESIAN_POINT('Origin',(0.,-0.75,1.3));
#19376=CARTESIAN_POINT('',(0.,-0.75,1.3));
#19377=CARTESIAN_POINT('',(0.,-0.75,1.3));
#19378=CARTESIAN_POINT('',(22.,-0.75,1.3));
#19379=CARTESIAN_POINT('',(22.,-0.75,1.3));
#19380=CARTESIAN_POINT('',(0.,-0.75,1.3));
#19381=CARTESIAN_POINT('Origin',(0.,-0.75,1.5));
#19382=CARTESIAN_POINT('',(0.,-0.75,1.5));
#19383=CARTESIAN_POINT('',(0.,-0.75,1.5));
#19384=CARTESIAN_POINT('',(22.,-0.75,1.5));
#19385=CARTESIAN_POINT('',(22.,-0.75,1.5));
#19386=CARTESIAN_POINT('',(0.,-0.75,1.5));
#19387=CARTESIAN_POINT('Origin',(0.,0.75,1.5));
#19388=CARTESIAN_POINT('',(0.,0.75,1.5));
#19389=CARTESIAN_POINT('',(0.,0.75,1.5));
#19390=CARTESIAN_POINT('',(22.,0.75,1.5));
#19391=CARTESIAN_POINT('',(22.,0.75,1.5));
#19392=CARTESIAN_POINT('',(0.,0.75,1.5));
#19393=CARTESIAN_POINT('Origin',(0.,0.75,1.3));
#19394=CARTESIAN_POINT('',(0.,0.75,1.3));
#19395=CARTESIAN_POINT('',(0.,0.75,1.3));
#19396=CARTESIAN_POINT('',(22.,0.75,1.3));
#19397=CARTESIAN_POINT('',(22.,0.75,1.3));
#19398=CARTESIAN_POINT('',(0.,0.75,1.3));
#19399=CARTESIAN_POINT('Origin',(0.,0.53,1.15));
#19400=CARTESIAN_POINT('',(0.,0.53,1.15));
#19401=CARTESIAN_POINT('',(0.,0.53,1.15));
#19402=CARTESIAN_POINT('',(22.,0.53,1.15));
#19403=CARTESIAN_POINT('',(22.,0.53,1.15));
#19404=CARTESIAN_POINT('',(0.,0.53,1.15));
#19405=CARTESIAN_POINT('Origin',(0.,0.53,1.));
#19406=CARTESIAN_POINT('',(0.,0.53,1.));
#19407=CARTESIAN_POINT('',(0.,0.53,1.));
#19408=CARTESIAN_POINT('',(22.,0.53,1.));
#19409=CARTESIAN_POINT('',(22.,0.53,1.));
#19410=CARTESIAN_POINT('',(0.,0.53,1.));
#19411=CARTESIAN_POINT('Origin',(0.,0.75,0.85));
#19412=CARTESIAN_POINT('',(0.,0.75,0.85));
#19413=CARTESIAN_POINT('',(0.,0.75,0.85));
#19414=CARTESIAN_POINT('',(22.,0.75,0.85));
#19415=CARTESIAN_POINT('',(22.,0.75,0.85));
#19416=CARTESIAN_POINT('',(0.,0.75,0.85));
#19417=CARTESIAN_POINT('Origin',(0.,0.75,0.));
#19418=CARTESIAN_POINT('',(0.,0.75,0.));
#19419=CARTESIAN_POINT('',(0.,0.75,0.));
#19420=CARTESIAN_POINT('',(22.,0.75,0.));
#19421=CARTESIAN_POINT('',(22.,0.75,0.));
#19422=CARTESIAN_POINT('',(0.,0.75,0.));
#19423=CARTESIAN_POINT('Origin',(0.,-0.75,0.));
#19424=CARTESIAN_POINT('',(0.,-0.75,0.));
#19425=CARTESIAN_POINT('',(0.,-0.75,0.));
#19426=CARTESIAN_POINT('',(22.,-0.75,0.));
#19427=CARTESIAN_POINT('',(22.,-0.75,0.));
#19428=CARTESIAN_POINT('',(0.,-0.75,0.));
#19429=CARTESIAN_POINT('Origin',(0.,-0.75,0.85));
#19430=CARTESIAN_POINT('',(0.,-0.75,0.85));
#19431=CARTESIAN_POINT('',(22.,-0.75,0.85));
#19432=CARTESIAN_POINT('Origin',(22.,0.,0.75));
#19433=CARTESIAN_POINT('Origin',(0.,0.,0.75));
#23473=UNCERTAINTY_MEASURE_WITH_UNIT(LENGTH_MEASURE(0.001),#23588,
'DISTANCE_ACCURACY_VALUE',
'Maximum model space distance between geometric entities at asserted c
onnectivities');
#23522=UNCERTAINTY_MEASURE_WITH_UNIT(LENGTH_MEASURE(0.001),#23588,
'DISTANCE_ACCURACY_VALUE',
'Maximum model space distance between geometric entities at asserted c
onnectivities');
#23538=(
GEOMETRIC_REPRESENTATION_CONTEXT(3)
GLOBAL_UNCERTAINTY_ASSIGNED_CONTEXT((#23473))
GLOBAL_UNIT_ASSIGNED_CONTEXT((#23588,#23590,#23591))
REPRESENTATION_CONTEXT('','3D')
);
#23587=(
GEOMETRIC_REPRESENTATION_CONTEXT(3)
GLOBAL_UNCERTAINTY_ASSIGNED_CONTEXT((#23522))
GLOBAL_UNIT_ASSIGNED_CONTEXT((#23588,#23590,#23591))
REPRESENTATION_CONTEXT('','3D')
);
#23588=(
LENGTH_UNIT()
NAMED_UNIT(*)
SI_UNIT(.CENTI.,.METRE.)
);
#23590=(
NAMED_UNIT(*)
PLANE_ANGLE_UNIT()
SI_UNIT($,.RADIAN.)
);
#23591=(
NAMED_UNIT(*)
SI_UNIT($,.STERADIAN.)
SOLID_ANGLE_UNIT()
);
#23607=SHAPE_DEFINITION_REPRESENTATION(#23671,#23840);
#23671=PRODUCT_DEFINITION_SHAPE('',$,#23905);
#23840=SHAPE_REPRESENTATION('',(#13178),#23538);
#23889=PRODUCT_DEFINITION_CONTEXT('part definition',#24083,'design');
#23905=PRODUCT_DEFINITION('Linear Guide Rail - 15 mm, 220 mm Long',
'Linear Guide Rail - 15 mm, 220 mm Long',#23969,#23889);
#23969=PRODUCT_DEFINITION_FORMATION('',$,#24100);
#24083=APPLICATION_CONTEXT(
'Core Data for Automotive Mechanical Design Process');
#24084=PRODUCT_CONTEXT('part definition',#24083,'mechanical');
#24100=PRODUCT('Linear Guide Rail - 15 mm, 220 mm Long',
'Linear Guide Rail - 15 mm, 220 mm Long',
'Linear Guide Rail - 15 mm, 220 mm Long',(#24084));
#24198=COLOUR_RGB('Sky Blue',0.24,0.69,0.87);
#24199=FILL_AREA_STYLE_COLOUR('',#24198);
#24200=FILL_AREA_STYLE('',(#24199));
#24201=SURFACE_STYLE_FILL_AREA(#24200);
#24202=SURFACE_SIDE_STYLE('',(#24201));
#24203=SURFACE_STYLE_USAGE(.BOTH.,#24202);
#24204=PRESENTATION_STYLE_ASSIGNMENT((#24203));
ENDSEC;
END-ISO-10303-21;
